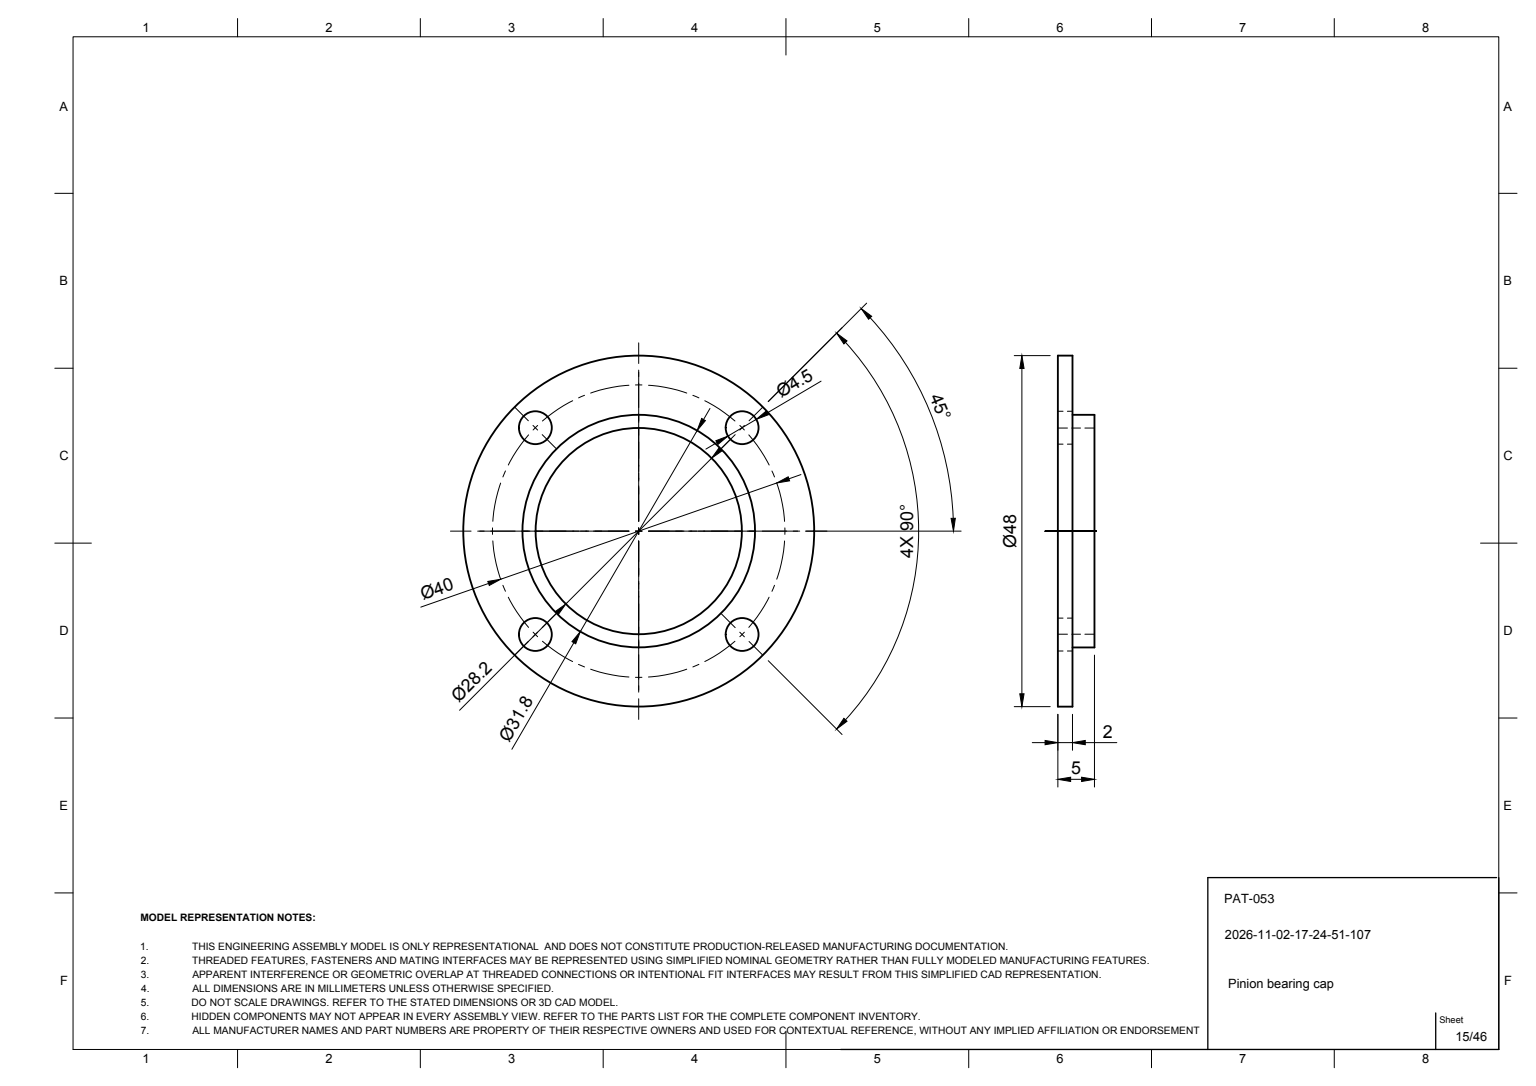
ISO-10303-21;
HEADER;
/* Generated by software containing ST-Developer
 * from STEP Tools, Inc. (www.steptools.com) 
 */

FILE_DESCRIPTION(
/* description */ ('Hand-operated arbor press'),
/* implementation_level */ '2;1');

FILE_NAME(
/* name */ 'Pinion bearing cap.step',
/* time_stamp */ '2026-10-28T03:25:25-07:00',
/* author */ (''),
/* organization */ (''),
/* preprocessor_version */ 'ST-DEVELOPER v20.2',
/* originating_system */ 'Autodesk Translation Framework v15.17.0.0',
/* authorisation */ '');

FILE_SCHEMA (('AUTOMOTIVE_DESIGN { 1 0 10303 214 3 1 1 }'));
ENDSEC;

DATA;
#10=MECHANICAL_DESIGN_GEOMETRIC_PRESENTATION_REPRESENTATION('',(#596),#32751);
#512=SHAPE_REPRESENTATION_RELATIONSHIP('SRR','None',#32941,#554);
#554=ADVANCED_BREP_SHAPE_REPRESENTATION('',(#645),#32715);
#596=STYLED_ITEM('',(#33242),#645);
#645=MANIFOLD_SOLID_BREP('Body1',#12493);
#743=FACE_BOUND('',#2188,.T.);
#744=FACE_BOUND('',#2191,.T.);
#745=FACE_BOUND('',#2192,.T.);
#746=FACE_BOUND('',#2193,.T.);
#747=FACE_BOUND('',#2194,.T.);
#748=FACE_BOUND('',#2195,.T.);
#749=FACE_BOUND('',#2197,.T.);
#750=FACE_BOUND('',#2198,.T.);
#751=FACE_BOUND('',#2199,.T.);
#752=FACE_BOUND('',#2200,.T.);
#753=FACE_BOUND('',#2201,.T.);
#944=PLANE('',#13272);
#945=PLANE('',#13276);
#946=PLANE('',#13277);
#1437=FACE_OUTER_BOUND('',#2181,.T.);
#1438=FACE_OUTER_BOUND('',#2182,.T.);
#1439=FACE_OUTER_BOUND('',#2183,.T.);
#1440=FACE_OUTER_BOUND('',#2184,.T.);
#1441=FACE_OUTER_BOUND('',#2185,.T.);
#1442=FACE_OUTER_BOUND('',#2186,.T.);
#1443=FACE_OUTER_BOUND('',#2187,.T.);
#1444=FACE_OUTER_BOUND('',#2189,.T.);
#1445=FACE_OUTER_BOUND('',#2190,.T.);
#1446=FACE_OUTER_BOUND('',#2196,.T.);
#2181=EDGE_LOOP('',(#9014,#9015,#9016,#9017));
#2182=EDGE_LOOP('',(#9018,#9019,#9020,#9021));
#2183=EDGE_LOOP('',(#9022,#9023,#9024,#9025));
#2184=EDGE_LOOP('',(#9026,#9027,#9028,#9029));
#2185=EDGE_LOOP('',(#9030,#9031,#9032,#9033));
#2186=EDGE_LOOP('',(#9034,#9035,#9036,#9037));
#2187=EDGE_LOOP('',(#9038));
#2188=EDGE_LOOP('',(#9039));
#2189=EDGE_LOOP('',(#9040,#9041,#9042,#9043));
#2190=EDGE_LOOP('',(#9044));
#2191=EDGE_LOOP('',(#9045));
#2192=EDGE_LOOP('',(#9046));
#2193=EDGE_LOOP('',(#9047));
#2194=EDGE_LOOP('',(#9048));
#2195=EDGE_LOOP('',(#9049));
#2196=EDGE_LOOP('',(#9050));
#2197=EDGE_LOOP('',(#9051));
#2198=EDGE_LOOP('',(#9052));
#2199=EDGE_LOOP('',(#9053));
#2200=EDGE_LOOP('',(#9054));
#2201=EDGE_LOOP('',(#9055));
#3071=LINE('',#18374,#4242);
#3072=LINE('',#18380,#4243);
#3073=LINE('',#18386,#4244);
#3074=LINE('',#18392,#4245);
#3075=LINE('',#18398,#4246);
#3076=LINE('',#18404,#4247);
#3077=LINE('',#18411,#4248);
#4242=VECTOR('',#14916,1.41);
#4243=VECTOR('',#14923,0.225);
#4244=VECTOR('',#14930,0.225);
#4245=VECTOR('',#14937,0.225);
#4246=VECTOR('',#14944,0.225);
#4247=VECTOR('',#14951,1.59);
#4248=VECTOR('',#14960,2.4);
#5264=CIRCLE('',#13255,1.41);
#5265=CIRCLE('',#13256,1.41);
#5266=CIRCLE('',#13258,0.225);
#5267=CIRCLE('',#13259,0.225);
#5268=CIRCLE('',#13261,0.225);
#5269=CIRCLE('',#13262,0.225);
#5270=CIRCLE('',#13264,0.225);
#5271=CIRCLE('',#13265,0.225);
#5272=CIRCLE('',#13267,0.225);
#5273=CIRCLE('',#13268,0.225);
#5274=CIRCLE('',#13270,1.59);
#5275=CIRCLE('',#13271,1.59);
#5276=CIRCLE('',#13274,2.4);
#5277=CIRCLE('',#13275,2.4);
#5786=VERTEX_POINT('',#18371);
#5787=VERTEX_POINT('',#18373);
#5788=VERTEX_POINT('',#18377);
#5789=VERTEX_POINT('',#18379);
#5790=VERTEX_POINT('',#18383);
#5791=VERTEX_POINT('',#18385);
#5792=VERTEX_POINT('',#18389);
#5793=VERTEX_POINT('',#18391);
#5794=VERTEX_POINT('',#18395);
#5795=VERTEX_POINT('',#18397);
#5796=VERTEX_POINT('',#18401);
#5797=VERTEX_POINT('',#18403);
#5798=VERTEX_POINT('',#18408);
#5799=VERTEX_POINT('',#18410);
#7010=EDGE_CURVE('',#5786,#5786,#5264,.T.);
#7011=EDGE_CURVE('',#5786,#5787,#3071,.T.);
#7012=EDGE_CURVE('',#5787,#5787,#5265,.T.);
#7013=EDGE_CURVE('',#5788,#5788,#5266,.T.);
#7014=EDGE_CURVE('',#5788,#5789,#3072,.T.);
#7015=EDGE_CURVE('',#5789,#5789,#5267,.T.);
#7016=EDGE_CURVE('',#5790,#5790,#5268,.T.);
#7017=EDGE_CURVE('',#5790,#5791,#3073,.T.);
#7018=EDGE_CURVE('',#5791,#5791,#5269,.T.);
#7019=EDGE_CURVE('',#5792,#5792,#5270,.T.);
#7020=EDGE_CURVE('',#5792,#5793,#3074,.T.);
#7021=EDGE_CURVE('',#5793,#5793,#5271,.T.);
#7022=EDGE_CURVE('',#5794,#5794,#5272,.T.);
#7023=EDGE_CURVE('',#5794,#5795,#3075,.T.);
#7024=EDGE_CURVE('',#5795,#5795,#5273,.T.);
#7025=EDGE_CURVE('',#5796,#5796,#5274,.T.);
#7026=EDGE_CURVE('',#5796,#5797,#3076,.T.);
#7027=EDGE_CURVE('',#5797,#5797,#5275,.T.);
#7028=EDGE_CURVE('',#5798,#5798,#5276,.T.);
#7029=EDGE_CURVE('',#5798,#5799,#3077,.T.);
#7030=EDGE_CURVE('',#5799,#5799,#5277,.T.);
#9014=ORIENTED_EDGE('',*,*,#7010,.F.);
#9015=ORIENTED_EDGE('',*,*,#7011,.T.);
#9016=ORIENTED_EDGE('',*,*,#7012,.F.);
#9017=ORIENTED_EDGE('',*,*,#7011,.F.);
#9018=ORIENTED_EDGE('',*,*,#7013,.F.);
#9019=ORIENTED_EDGE('',*,*,#7014,.T.);
#9020=ORIENTED_EDGE('',*,*,#7015,.F.);
#9021=ORIENTED_EDGE('',*,*,#7014,.F.);
#9022=ORIENTED_EDGE('',*,*,#7016,.F.);
#9023=ORIENTED_EDGE('',*,*,#7017,.T.);
#9024=ORIENTED_EDGE('',*,*,#7018,.F.);
#9025=ORIENTED_EDGE('',*,*,#7017,.F.);
#9026=ORIENTED_EDGE('',*,*,#7019,.F.);
#9027=ORIENTED_EDGE('',*,*,#7020,.T.);
#9028=ORIENTED_EDGE('',*,*,#7021,.F.);
#9029=ORIENTED_EDGE('',*,*,#7020,.F.);
#9030=ORIENTED_EDGE('',*,*,#7022,.F.);
#9031=ORIENTED_EDGE('',*,*,#7023,.T.);
#9032=ORIENTED_EDGE('',*,*,#7024,.F.);
#9033=ORIENTED_EDGE('',*,*,#7023,.F.);
#9034=ORIENTED_EDGE('',*,*,#7025,.F.);
#9035=ORIENTED_EDGE('',*,*,#7026,.T.);
#9036=ORIENTED_EDGE('',*,*,#7027,.F.);
#9037=ORIENTED_EDGE('',*,*,#7026,.F.);
#9038=ORIENTED_EDGE('',*,*,#7025,.T.);
#9039=ORIENTED_EDGE('',*,*,#7012,.T.);
#9040=ORIENTED_EDGE('',*,*,#7028,.F.);
#9041=ORIENTED_EDGE('',*,*,#7029,.T.);
#9042=ORIENTED_EDGE('',*,*,#7030,.T.);
#9043=ORIENTED_EDGE('',*,*,#7029,.F.);
#9044=ORIENTED_EDGE('',*,*,#7028,.T.);
#9045=ORIENTED_EDGE('',*,*,#7027,.T.);
#9046=ORIENTED_EDGE('',*,*,#7024,.T.);
#9047=ORIENTED_EDGE('',*,*,#7021,.T.);
#9048=ORIENTED_EDGE('',*,*,#7018,.T.);
#9049=ORIENTED_EDGE('',*,*,#7015,.T.);
#9050=ORIENTED_EDGE('',*,*,#7030,.F.);
#9051=ORIENTED_EDGE('',*,*,#7010,.T.);
#9052=ORIENTED_EDGE('',*,*,#7022,.T.);
#9053=ORIENTED_EDGE('',*,*,#7019,.T.);
#9054=ORIENTED_EDGE('',*,*,#7016,.T.);
#9055=ORIENTED_EDGE('',*,*,#7013,.T.);
#11691=CYLINDRICAL_SURFACE('',#13254,1.41);
#11692=CYLINDRICAL_SURFACE('',#13257,0.225);
#11693=CYLINDRICAL_SURFACE('',#13260,0.225);
#11694=CYLINDRICAL_SURFACE('',#13263,0.225);
#11695=CYLINDRICAL_SURFACE('',#13266,0.225);
#11696=CYLINDRICAL_SURFACE('',#13269,1.59);
#11697=CYLINDRICAL_SURFACE('',#13273,2.4);
#11946=ADVANCED_FACE('',(#1437),#11691,.F.);
#11947=ADVANCED_FACE('',(#1438),#11692,.F.);
#11948=ADVANCED_FACE('',(#1439),#11693,.F.);
#11949=ADVANCED_FACE('',(#1440),#11694,.F.);
#11950=ADVANCED_FACE('',(#1441),#11695,.F.);
#11951=ADVANCED_FACE('',(#1442),#11696,.T.);
#11952=ADVANCED_FACE('',(#1443,#743),#944,.T.);
#11953=ADVANCED_FACE('',(#1444),#11697,.T.);
#11954=ADVANCED_FACE('',(#1445,#744,#745,#746,#747,#748),#945,.T.);
#11955=ADVANCED_FACE('',(#1446,#749,#750,#751,#752,#753),#946,.F.);
#12493=CLOSED_SHELL('',(#11946,#11947,#11948,#11949,#11950,#11951,#11952,
#11953,#11954,#11955));
#13253=AXIS2_PLACEMENT_3D('',#18369,#14910,#14911);
#13254=AXIS2_PLACEMENT_3D('',#18370,#14912,#14913);
#13255=AXIS2_PLACEMENT_3D('',#18372,#14914,#14915);
#13256=AXIS2_PLACEMENT_3D('',#18375,#14917,#14918);
#13257=AXIS2_PLACEMENT_3D('',#18376,#14919,#14920);
#13258=AXIS2_PLACEMENT_3D('',#18378,#14921,#14922);
#13259=AXIS2_PLACEMENT_3D('',#18381,#14924,#14925);
#13260=AXIS2_PLACEMENT_3D('',#18382,#14926,#14927);
#13261=AXIS2_PLACEMENT_3D('',#18384,#14928,#14929);
#13262=AXIS2_PLACEMENT_3D('',#18387,#14931,#14932);
#13263=AXIS2_PLACEMENT_3D('',#18388,#14933,#14934);
#13264=AXIS2_PLACEMENT_3D('',#18390,#14935,#14936);
#13265=AXIS2_PLACEMENT_3D('',#18393,#14938,#14939);
#13266=AXIS2_PLACEMENT_3D('',#18394,#14940,#14941);
#13267=AXIS2_PLACEMENT_3D('',#18396,#14942,#14943);
#13268=AXIS2_PLACEMENT_3D('',#18399,#14945,#14946);
#13269=AXIS2_PLACEMENT_3D('',#18400,#14947,#14948);
#13270=AXIS2_PLACEMENT_3D('',#18402,#14949,#14950);
#13271=AXIS2_PLACEMENT_3D('',#18405,#14952,#14953);
#13272=AXIS2_PLACEMENT_3D('',#18406,#14954,#14955);
#13273=AXIS2_PLACEMENT_3D('',#18407,#14956,#14957);
#13274=AXIS2_PLACEMENT_3D('',#18409,#14958,#14959);
#13275=AXIS2_PLACEMENT_3D('',#18412,#14961,#14962);
#13276=AXIS2_PLACEMENT_3D('',#18413,#14963,#14964);
#13277=AXIS2_PLACEMENT_3D('',#18414,#14965,#14966);
#14910=DIRECTION('axis',(0.,0.,1.));
#14911=DIRECTION('refdir',(1.,0.,0.));
#14912=DIRECTION('center_axis',(0.,1.,0.));
#14913=DIRECTION('ref_axis',(1.,0.,0.));
#14914=DIRECTION('center_axis',(0.,1.,0.));
#14915=DIRECTION('ref_axis',(1.,0.,0.));
#14916=DIRECTION('',(0.,1.,0.));
#14917=DIRECTION('center_axis',(0.,-1.,0.));
#14918=DIRECTION('ref_axis',(1.,0.,0.));
#14919=DIRECTION('center_axis',(0.,1.,0.));
#14920=DIRECTION('ref_axis',(1.,0.,0.));
#14921=DIRECTION('center_axis',(0.,1.,0.));
#14922=DIRECTION('ref_axis',(1.,0.,0.));
#14923=DIRECTION('',(0.,1.,0.));
#14924=DIRECTION('center_axis',(0.,-1.,0.));
#14925=DIRECTION('ref_axis',(1.,0.,0.));
#14926=DIRECTION('center_axis',(0.,1.,0.));
#14927=DIRECTION('ref_axis',(1.,0.,0.));
#14928=DIRECTION('center_axis',(0.,1.,0.));
#14929=DIRECTION('ref_axis',(1.,0.,0.));
#14930=DIRECTION('',(0.,1.,0.));
#14931=DIRECTION('center_axis',(0.,-1.,0.));
#14932=DIRECTION('ref_axis',(1.,0.,0.));
#14933=DIRECTION('center_axis',(0.,1.,0.));
#14934=DIRECTION('ref_axis',(1.,0.,0.));
#14935=DIRECTION('center_axis',(0.,1.,0.));
#14936=DIRECTION('ref_axis',(1.,0.,0.));
#14937=DIRECTION('',(0.,1.,0.));
#14938=DIRECTION('center_axis',(0.,-1.,0.));
#14939=DIRECTION('ref_axis',(1.,0.,0.));
#14940=DIRECTION('center_axis',(0.,1.,0.));
#14941=DIRECTION('ref_axis',(1.,0.,0.));
#14942=DIRECTION('center_axis',(0.,1.,0.));
#14943=DIRECTION('ref_axis',(1.,0.,0.));
#14944=DIRECTION('',(0.,1.,0.));
#14945=DIRECTION('center_axis',(0.,-1.,0.));
#14946=DIRECTION('ref_axis',(1.,0.,0.));
#14947=DIRECTION('center_axis',(0.,1.,0.));
#14948=DIRECTION('ref_axis',(1.,0.,0.));
#14949=DIRECTION('center_axis',(0.,1.,0.));
#14950=DIRECTION('ref_axis',(1.,0.,0.));
#14951=DIRECTION('',(0.,-1.,0.));
#14952=DIRECTION('center_axis',(0.,-1.,0.));
#14953=DIRECTION('ref_axis',(1.,0.,0.));
#14954=DIRECTION('center_axis',(0.,1.,0.));
#14955=DIRECTION('ref_axis',(1.,0.,0.));
#14956=DIRECTION('center_axis',(0.,1.,0.));
#14957=DIRECTION('ref_axis',(1.,0.,0.));
#14958=DIRECTION('center_axis',(0.,1.,0.));
#14959=DIRECTION('ref_axis',(1.,0.,0.));
#14960=DIRECTION('',(0.,-1.,0.));
#14961=DIRECTION('center_axis',(0.,1.,0.));
#14962=DIRECTION('ref_axis',(1.,0.,0.));
#14963=DIRECTION('center_axis',(0.,1.,0.));
#14964=DIRECTION('ref_axis',(1.,0.,0.));
#14965=DIRECTION('center_axis',(0.,1.,0.));
#14966=DIRECTION('ref_axis',(1.,0.,0.));
#18369=CARTESIAN_POINT('',(0.,0.,0.));
#18370=CARTESIAN_POINT('Origin',(-3.25,-4.1,20.));
#18371=CARTESIAN_POINT('',(-4.66,-4.,20.));
#18372=CARTESIAN_POINT('Origin',(-3.25,-4.,20.));
#18373=CARTESIAN_POINT('',(-4.66,-3.5,20.));
#18374=CARTESIAN_POINT('',(-4.66,-4.1,20.));
#18375=CARTESIAN_POINT('Origin',(-3.25,-3.5,20.));
#18376=CARTESIAN_POINT('Origin',(-4.66421356237309,-4.1,18.5857864376269));
#18377=CARTESIAN_POINT('',(-4.88921356237309,-4.,18.5857864376269));
#18378=CARTESIAN_POINT('Origin',(-4.66421356237309,-4.,18.5857864376269));
#18379=CARTESIAN_POINT('',(-4.88921356237309,-3.8,18.5857864376269));
#18380=CARTESIAN_POINT('',(-4.88921356237309,-4.1,18.5857864376269));
#18381=CARTESIAN_POINT('Origin',(-4.66421356237309,-3.8,18.5857864376269));
#18382=CARTESIAN_POINT('Origin',(-4.66421356237309,-4.1,21.4142135623731));
#18383=CARTESIAN_POINT('',(-4.88921356237309,-4.,21.4142135623731));
#18384=CARTESIAN_POINT('Origin',(-4.66421356237309,-4.,21.4142135623731));
#18385=CARTESIAN_POINT('',(-4.88921356237309,-3.8,21.4142135623731));
#18386=CARTESIAN_POINT('',(-4.88921356237309,-4.1,21.4142135623731));
#18387=CARTESIAN_POINT('Origin',(-4.66421356237309,-3.8,21.4142135623731));
#18388=CARTESIAN_POINT('Origin',(-1.8357864376269,-4.1,21.4142135623731));
#18389=CARTESIAN_POINT('',(-2.0607864376269,-4.,21.4142135623731));
#18390=CARTESIAN_POINT('Origin',(-1.8357864376269,-4.,21.4142135623731));
#18391=CARTESIAN_POINT('',(-2.0607864376269,-3.8,21.4142135623731));
#18392=CARTESIAN_POINT('',(-2.0607864376269,-4.1,21.4142135623731));
#18393=CARTESIAN_POINT('Origin',(-1.8357864376269,-3.8,21.4142135623731));
#18394=CARTESIAN_POINT('Origin',(-1.83578643762691,-4.1,18.5857864376269));
#18395=CARTESIAN_POINT('',(-2.06078643762691,-4.,18.5857864376269));
#18396=CARTESIAN_POINT('Origin',(-1.83578643762691,-4.,18.5857864376269));
#18397=CARTESIAN_POINT('',(-2.06078643762691,-3.8,18.5857864376269));
#18398=CARTESIAN_POINT('',(-2.06078643762691,-4.1,18.5857864376269));
#18399=CARTESIAN_POINT('Origin',(-1.83578643762691,-3.8,18.5857864376269));
#18400=CARTESIAN_POINT('Origin',(-3.25,-3.8,20.));
#18401=CARTESIAN_POINT('',(-4.84,-3.5,20.));
#18402=CARTESIAN_POINT('Origin',(-3.25,-3.5,20.));
#18403=CARTESIAN_POINT('',(-4.84,-3.8,20.));
#18404=CARTESIAN_POINT('',(-4.84,-3.8,20.));
#18405=CARTESIAN_POINT('Origin',(-3.25,-3.8,20.));
#18406=CARTESIAN_POINT('Origin',(-3.25,-3.5,20.));
#18407=CARTESIAN_POINT('Origin',(-3.25,-4.,20.));
#18408=CARTESIAN_POINT('',(-5.65,-3.8,20.));
#18409=CARTESIAN_POINT('Origin',(-3.25,-3.8,20.));
#18410=CARTESIAN_POINT('',(-5.65,-4.,20.));
#18411=CARTESIAN_POINT('',(-5.65,-4.,20.));
#18412=CARTESIAN_POINT('Origin',(-3.25,-4.,20.));
#18413=CARTESIAN_POINT('Origin',(-3.25,-3.8,20.));
#18414=CARTESIAN_POINT('Origin',(-3.25,-4.,20.));
#32666=UNCERTAINTY_MEASURE_WITH_UNIT(LENGTH_MEASURE(0.001),#32752,
'DISTANCE_ACCURACY_VALUE',
'Maximum model space distance between geometric entities at asserted c
onnectivities');
#32702=UNCERTAINTY_MEASURE_WITH_UNIT(LENGTH_MEASURE(0.001),#32752,
'DISTANCE_ACCURACY_VALUE',
'Maximum model space distance between geometric entities at asserted c
onnectivities');
#32715=(
GEOMETRIC_REPRESENTATION_CONTEXT(3)
GLOBAL_UNCERTAINTY_ASSIGNED_CONTEXT((#32666))
GLOBAL_UNIT_ASSIGNED_CONTEXT((#32752,#32754,#32755))
REPRESENTATION_CONTEXT('','3D')
);
#32751=(
GEOMETRIC_REPRESENTATION_CONTEXT(3)
GLOBAL_UNCERTAINTY_ASSIGNED_CONTEXT((#32702))
GLOBAL_UNIT_ASSIGNED_CONTEXT((#32752,#32754,#32755))
REPRESENTATION_CONTEXT('','3D')
);
#32752=(
LENGTH_UNIT()
NAMED_UNIT(*)
SI_UNIT(.CENTI.,.METRE.)
);
#32754=(
NAMED_UNIT(*)
PLANE_ANGLE_UNIT()
SI_UNIT($,.RADIAN.)
);
#32755=(
NAMED_UNIT(*)
SI_UNIT($,.STERADIAN.)
SOLID_ANGLE_UNIT()
);
#32768=SHAPE_DEFINITION_REPRESENTATION(#32816,#32941);
#32816=PRODUCT_DEFINITION_SHAPE('',$,#32990);
#32941=SHAPE_REPRESENTATION('',(#13253),#32715);
#32977=PRODUCT_DEFINITION_CONTEXT('part definition',#33123,'design');
#32990=PRODUCT_DEFINITION('Pinion bearing cap','Pinion bearing cap',#33038,
#32977);
#33038=PRODUCT_DEFINITION_FORMATION('',$,#33137);
#33123=APPLICATION_CONTEXT(
'Core Data for Automotive Mechanical Design Process');
#33124=PRODUCT_CONTEXT('part definition',#33123,'mechanical');
#33137=PRODUCT('Pinion bearing cap','Pinion bearing cap',
'Pinion bearing cap',(#33124));
#33236=COLOUR_RGB('Grey',0.48,0.52,0.57);
#33237=FILL_AREA_STYLE_COLOUR('',#33236);
#33238=FILL_AREA_STYLE('',(#33237));
#33239=SURFACE_STYLE_FILL_AREA(#33238);
#33240=SURFACE_SIDE_STYLE('',(#33239));
#33241=SURFACE_STYLE_USAGE(.BOTH.,#33240);
#33242=PRESENTATION_STYLE_ASSIGNMENT((#33241));
ENDSEC;
END-ISO-10303-21;
